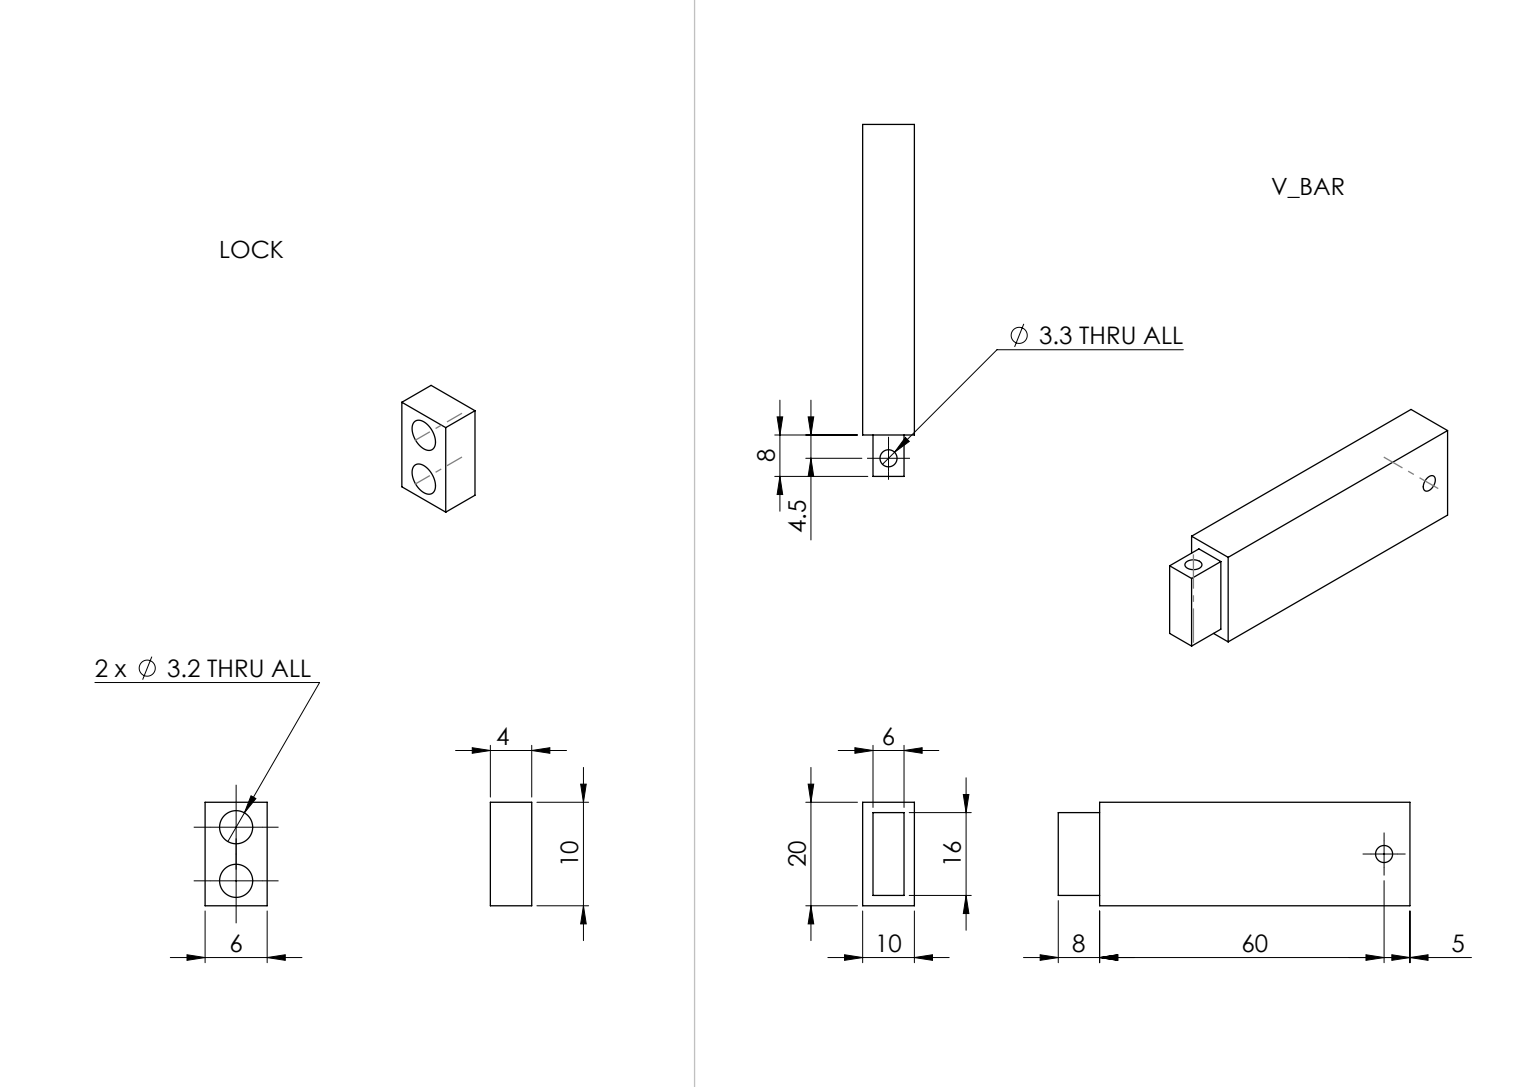
ISO-10303-21;
HEADER;
FILE_DESCRIPTION (('STEP AP214'),
    '1' );
FILE_NAME ('V_bar.step',
    '2026-10-08T12:12:07',
    ( '' ),
    ( '' ),
    'SwSTEP 2.0',
    'SolidWorks 2026',
    '' );
FILE_SCHEMA (( 'AUTOMOTIVE_DESIGN' ));
ENDSEC;

DATA;
#54=CARTESIAN_POINT ( 'NONE',  ( 55.00000000000000000, -8.000000000000001776, -4.499999999999986677 ) ) ;
#92=( NAMED_UNIT ( * ) PLANE_ANGLE_UNIT ( ) SI_UNIT ( $, .RADIAN. ) );
#93=AXIS2_PLACEMENT_3D ( 'NONE', #1716, #4922, #1673 ) ;
#102=VECTOR ( 'NONE', #7211, 1000.000000000000000 ) ;
#104=VECTOR ( 'NONE', #3751, 1000.000000000000000 ) ;
#145=LINE ( 'NONE', #2653, #909 ) ;
#163=DIRECTION ( 'NONE',  ( 0.000000000000000000, 1.000000000000000000, -0.000000000000000000 ) ) ;
#215=DIRECTION ( 'NONE',  ( 0.000000000000000000, 0.000000000000000000, 1.000000000000000000 ) ) ;
#229=ORIENTED_EDGE ( 'NONE', *, *, #6061, .F. ) ;
#234=LINE ( 'NONE', #6015, #2684 ) ;
#235=PLANE ( 'NONE',  #5820 ) ;
#258=DIRECTION ( 'NONE',  ( -0.000000000000000000, -1.000000000000000000, -0.000000000000000000 ) ) ;
#265=CARTESIAN_POINT ( 'NONE',  ( 60.00000000000000711, 9.332579536216795825E-15, 53.34999999999999432 ) ) ;
#266=CARTESIAN_POINT ( 'NONE',  ( 55.00000000000000000, 8.000000000000000000, -4.499999999999986677 ) ) ;
#270=CARTESIAN_POINT ( 'NONE',  ( 0.000000000000000000, 0.000000000000000000, 60.00000000000000000 ) ) ;
#293=ADVANCED_BREP_SHAPE_REPRESENTATION ( '', ( #1362, #1587 ), #1923 ) ;
#299=DIRECTION ( 'NONE',  ( 0.000000000000000000, 0.000000000000000000, -1.000000000000000000 ) ) ;
#302=FACE_BOUND ( 'NONE', #1666, .T. ) ;
#303=EDGE_CURVE ( 'NONE', #972, #4432, #3116, .T. ) ;
#319=LINE ( 'NONE', #2908, #3181 ) ;
#354=EDGE_CURVE ( 'NONE', #3615, #8148, #1959, .T. ) ;
#394=DIRECTION ( 'NONE',  ( 0.000000000000000000, 0.000000000000000000, 1.000000000000000000 ) ) ;
#407=DIRECTION ( 'NONE',  ( -0.000000000000000000, 1.000000000000000000, -0.000000000000000000 ) ) ;
#421=ORIENTED_EDGE ( 'NONE', *, *, #7234, .F. ) ;
#445=ADVANCED_FACE ( 'NONE', ( #302, #3325 ), #3433, .F. ) ;
#483=CARTESIAN_POINT ( 'NONE',  ( 50.00000000000000000, 9.332579536216795825E-15, 53.34999999999998010 ) ) ;
#539=CARTESIAN_POINT ( 'NONE',  ( 52.00000000000000711, -8.000000000000000000, -8.000000000000000000 ) ) ;
#555=CARTESIAN_POINT ( 'NONE',  ( 60.00000000000000711, 9.332579536216795825E-15, 54.99999999999997868 ) ) ;
#556=EDGE_CURVE ( 'NONE', #3047, #4432, #4306, .T. ) ;
#577=FACE_OUTER_BOUND ( 'NONE', #3634, .T. ) ;
#584=ORIENTED_EDGE ( 'NONE', *, *, #7801, .T. ) ;
#599=( LENGTH_UNIT ( ) NAMED_UNIT ( * ) SI_UNIT ( .MILLI., .METRE. ) );
#603=EDGE_LOOP ( 'NONE', ( #3185, #4958, #6458, #2037 ) ) ;
#684=DIRECTION ( 'NONE',  ( 0.000000000000000000, -1.000000000000000000, 0.000000000000000000 ) ) ;
#712=DIRECTION ( 'NONE',  ( 1.000000000000000000, -0.000000000000000000, -0.000000000000000000 ) ) ;
#717=ORIENTED_EDGE ( 'NONE', *, *, #2095, .F. ) ;
#723=SURFACE_STYLE_USAGE ( .BOTH. , #1946 ) ;
#724=AXIS2_PLACEMENT_3D ( 'NONE', #6540, #847, #215 ) ;
#726=FACE_OUTER_BOUND ( 'NONE', #4926, .T. ) ;
#743=DIRECTION ( 'NONE',  ( 0.000000000000000000, 0.000000000000000000, 1.000000000000000000 ) ) ;
#748=ORIENTED_EDGE ( 'NONE', *, *, #354, .T. ) ;
#760=AXIS2_PLACEMENT_3D ( 'NONE', #3959, #712, #2125 ) ;
#787=CARTESIAN_POINT ( 'NONE',  ( 60.00000000000000711, -10.00000000000000000, 60.00000000000000000 ) ) ;
#817=ORIENTED_EDGE ( 'NONE', *, *, #1983, .F. ) ;
#847=DIRECTION ( 'NONE',  ( 0.000000000000000000, 1.000000000000000000, -0.000000000000000000 ) ) ;
#879=CARTESIAN_POINT ( 'NONE',  ( 50.00000000000000000, -10.00000000000000000, 60.00000000000000000 ) ) ;
#897=EDGE_LOOP ( 'NONE', ( #2622, #3835 ) ) ;
#909=VECTOR ( 'NONE', #6307, 1000.000000000000000 ) ;
#916=VECTOR ( 'NONE', #3282, 1000.000000000000000 ) ;
#925=AXIS2_PLACEMENT_3D ( 'NONE', #4433, #1231, #6296 ) ;
#931=VERTEX_POINT ( 'NONE', #6838 ) ;
#942=EDGE_CURVE ( 'NONE', #8148, #2793, #145, .T. ) ;
#962=LINE ( 'NONE', #4254, #7895 ) ;
#972=VERTEX_POINT ( 'NONE', #2032 ) ;
#981=ORIENTED_EDGE ( 'NONE', *, *, #3877, .F. ) ;
#990=CARTESIAN_POINT ( 'NONE',  ( 50.00000000000000000, 10.00000000000000000, 60.00000000000000000 ) ) ;
#996=DIRECTION ( 'NONE',  ( 0.000000000000000000, 0.000000000000000000, -1.000000000000000000 ) ) ;
#1018=LINE ( 'NONE', #5356, #7945 ) ;
#1027=DIRECTION ( 'NONE',  ( 1.000000000000000000, 0.000000000000000000, 0.000000000000000000 ) ) ;
#1030=LINE ( 'NONE', #990, #5691 ) ;
#1046=ORIENTED_EDGE ( 'NONE', *, *, #7455, .T. ) ;
#1064=DIRECTION ( 'NONE',  ( 1.000000000000000000, 0.000000000000000000, 0.000000000000000000 ) ) ;
#1092=DIRECTION ( 'NONE',  ( 1.000000000000000000, -0.000000000000000000, -0.000000000000000000 ) ) ;
#1093=FILL_AREA_STYLE_COLOUR ( '', #7081 ) ;
#1106=STYLED_ITEM ( 'NONE', ( #5550 ), #293 ) ;
#1118=LINE ( 'NONE', #539, #4085 ) ;
#1136=( NAMED_UNIT ( * ) SI_UNIT ( $, .STERADIAN. ) SOLID_ANGLE_UNIT ( ) );
#1147=ORIENTED_EDGE ( 'NONE', *, *, #5934, .F. ) ;
#1162=ORIENTED_EDGE ( 'NONE', *, *, #6234, .T. ) ;
#1174=ORIENTED_EDGE ( 'NONE', *, *, #1998, .F. ) ;
#1193=AXIS2_PLACEMENT_3D ( 'NONE', #1933, #5753, #5667 ) ;
#1200=LINE ( 'NONE', #6929, #6572 ) ;
#1229=FILL_AREA_STYLE ('',( #1093 ) ) ;
#1231=DIRECTION ( 'NONE',  ( 1.000000000000000000, -0.000000000000000000, -0.000000000000000000 ) ) ;
#1248=DIRECTION ( 'NONE',  ( 0.000000000000000000, 1.000000000000000000, -0.000000000000000000 ) ) ;
#1277=EDGE_CURVE ( 'NONE', #5489, #8148, #8025, .T. ) ;
#1362=MANIFOLD_SOLID_BREP ( 'Tap Drill for M4 Tap2', #4092 ) ;
#1364=DIRECTION ( 'NONE',  ( 0.000000000000000000, -0.000000000000000000, 1.000000000000000000 ) ) ;
#1365=DIRECTION ( 'NONE',  ( 0.000000000000000000, 0.000000000000000000, 1.000000000000000000 ) ) ;
#1369=EDGE_CURVE ( 'NONE', #6012, #4327, #5321, .T. ) ;
#1390=FACE_BOUND ( 'NONE', #897, .T. ) ;
#1407=ORIENTED_EDGE ( 'NONE', *, *, #303, .F. ) ;
#1469=EDGE_CURVE ( 'NONE', #3630, #3047, #962, .T. ) ;
#1475=FACE_OUTER_BOUND ( 'NONE', #3870, .T. ) ;
#1486=DIRECTION ( 'NONE',  ( -1.000000000000000000, 0.000000000000000000, 0.000000000000000000 ) ) ;
#1507=CARTESIAN_POINT ( 'NONE',  ( 58.00000000000000000, -8.000000000000000000, 0.000000000000000000 ) ) ;
#1530=EDGE_LOOP ( 'NONE', ( #6903, #2912, #2180, #3251 ) ) ;
#1560=DIRECTION ( 'NONE',  ( 0.000000000000000000, 0.000000000000000000, 1.000000000000000000 ) ) ;
#1567=FACE_OUTER_BOUND ( 'NONE', #6558, .T. ) ;
#1587=AXIS2_PLACEMENT_3D ( 'NONE', #3942, #5152, #6454 ) ;
#1607=LINE ( 'NONE', #7781, #1909 ) ;
#1626=DIRECTION ( 'NONE',  ( -0.000000000000000000, -0.000000000000000000, -1.000000000000000000 ) ) ;
#1631=EDGE_CURVE ( 'NONE', #3615, #6597, #2117, .T. ) ;
#1658=CYLINDRICAL_SURFACE ( 'NONE', #5801, 1.649999999999995248 ) ;
#1663=CARTESIAN_POINT ( 'NONE',  ( 55.00000000000000000, 10.00000000000000000, -4.499999999999986677 ) ) ;
#1666=EDGE_LOOP ( 'NONE', ( #5675, #5495 ) ) ;
#1673=DIRECTION ( 'NONE',  ( 1.000000000000000000, 0.000000000000000000, -0.000000000000000000 ) ) ;
#1676=ORIENTED_EDGE ( 'NONE', *, *, #1631, .F. ) ;
#1704=VECTOR ( 'NONE', #6343, 1000.000000000000000 ) ;
#1709=VECTOR ( 'NONE', #7695, 1000.000000000000000 ) ;
#1714=ADVANCED_FACE ( 'NONE', ( #7304 ), #5443, .T. ) ;
#1716=CARTESIAN_POINT ( 'NONE',  ( 0.000000000000000000, 0.000000000000000000, -8.000000000000000000 ) ) ;
#1750=EDGE_CURVE ( 'NONE', #3287, #2510, #6633, .T. ) ;
#1753=CARTESIAN_POINT ( 'NONE',  ( 52.00000000000000711, -8.000000000000000000, -8.000000000000000000 ) ) ;
#1770=EDGE_CURVE ( 'NONE', #3287, #5411, #4813, .T. ) ;
#1785=ADVANCED_FACE ( 'NONE', ( #7339 ), #1658, .F. ) ;
#1828=EDGE_LOOP ( 'NONE', ( #2953, #1676, #6166, #1174 ) ) ;
#1840=ORIENTED_EDGE ( 'NONE', *, *, #1277, .F. ) ;
#1843=CARTESIAN_POINT ( 'NONE',  ( 58.00000000000000000, -8.000000000000000000, 0.000000000000000000 ) ) ;
#1876=PRODUCT ( 'V_bar', 'V_bar', '', ( #2708 ) ) ;
#1903=DIRECTION ( 'NONE',  ( 0.000000000000000000, 0.000000000000000000, -1.000000000000000000 ) ) ;
#1907=PRESENTATION_STYLE_ASSIGNMENT (( #723 ) ) ;
#1909=VECTOR ( 'NONE', #6570, 1000.000000000000000 ) ;
#1923=( GEOMETRIC_REPRESENTATION_CONTEXT ( 3 ) GLOBAL_UNCERTAINTY_ASSIGNED_CONTEXT ( ( #7447 ) ) GLOBAL_UNIT_ASSIGNED_CONTEXT ( ( #6567, #2842, #3508 ) ) REPRESENTATION_CONTEXT ( 'NONE', 'WORKASPACE' ) );
#1931=EDGE_LOOP ( 'NONE', ( #7376, #6911 ) ) ;
#1933=CARTESIAN_POINT ( 'NONE',  ( 60.00000000000000711, 10.00000000000000000, 60.00000000000000000 ) ) ;
#1946=SURFACE_SIDE_STYLE ('',( #6452 ) ) ;
#1956=VECTOR ( 'NONE', #6675, 1000.000000000000000 ) ;
#1959=LINE ( 'NONE', #2038, #2174 ) ;
#1983=EDGE_CURVE ( 'NONE', #4068, #4327, #1200, .T. ) ;
#1994=AXIS2_PLACEMENT_3D ( 'NONE', #7084, #1364, #5033 ) ;
#1998=EDGE_CURVE ( 'NONE', #7134, #931, #5155, .T. ) ;
#2032=CARTESIAN_POINT ( 'NONE',  ( 55.00000000000000000, -8.000000000000001776, -6.149999999999981704 ) ) ;
#2037=ORIENTED_EDGE ( 'NONE', *, *, #6966, .T. ) ;
#2038=CARTESIAN_POINT ( 'NONE',  ( 52.00000000000000711, 8.000000000000000000, -8.000000000000000000 ) ) ;
#2086=CARTESIAN_POINT ( 'NONE',  ( 50.00000000000000000, -10.00000000000000000, 60.00000000000000000 ) ) ;
#2090=ORIENTED_EDGE ( 'NONE', *, *, #1631, .T. ) ;
#2095=EDGE_CURVE ( 'NONE', #2510, #6841, #4753, .T. ) ;
#2111=AXIS2_PLACEMENT_3D ( 'NONE', #555, #3635, #6698 ) ;
#2117=LINE ( 'NONE', #5245, #3398 ) ;
#2121=CIRCLE ( 'NONE', #3049, 1.649999999999998579 ) ;
#2125=DIRECTION ( 'NONE',  ( 0.000000000000000000, 0.000000000000000000, -1.000000000000000000 ) ) ;
#2137=EDGE_CURVE ( 'NONE', #6584, #6037, #1607, .T. ) ;
#2174=VECTOR ( 'NONE', #5693, 1000.000000000000000 ) ;
#2180=ORIENTED_EDGE ( 'NONE', *, *, #5385, .T. ) ;
#2191=CARTESIAN_POINT ( 'NONE',  ( 55.00000000000000000, 10.00000000000000000, -4.499999999999986677 ) ) ;
#2192=EDGE_CURVE ( 'NONE', #4327, #6012, #4142, .T. ) ;
#2197=CARTESIAN_POINT ( 'NONE',  ( 50.00000000000000000, 10.00000000000000000, 60.00000000000000000 ) ) ;
#2281=ORIENTED_EDGE ( 'NONE', *, *, #4024, .T. ) ;
#2327=ORIENTED_EDGE ( 'NONE', *, *, #6061, .T. ) ;
#2335=AXIS2_PLACEMENT_3D ( 'NONE', #270, #7961, #4065 ) ;
#2360=PLANE ( 'NONE',  #6129 ) ;
#2361=VECTOR ( 'NONE', #7420, 1000.000000000000000 ) ;
#2362=LINE ( 'NONE', #3529, #7673 ) ;
#2376=PLANE ( 'NONE',  #93 ) ;
#2380=VECTOR ( 'NONE', #2938, 1000.000000000000000 ) ;
#2390=CARTESIAN_POINT ( 'NONE',  ( 58.00000000000000000, -8.000000000000000000, -8.000000000000000000 ) ) ;
#2423=CARTESIAN_POINT ( 'NONE',  ( 52.00000000000000711, 8.000000000000000000, -8.000000000000000000 ) ) ;
#2453=CARTESIAN_POINT ( 'NONE',  ( 60.00000000000000711, -10.00000000000000000, 0.000000000000000000 ) ) ;
#2466=ORIENTED_EDGE ( 'NONE', *, *, #3877, .T. ) ;
#2502=ORIENTED_EDGE ( 'NONE', *, *, #942, .F. ) ;
#2510=VERTEX_POINT ( 'NONE', #2197 ) ;
#2520=EDGE_CURVE ( 'NONE', #2793, #5096, #234, .T. ) ;
#2537=COLOUR_RGB ( '', 0.66274510, 0.83137255, 0.94901961) ;
#2592=ADVANCED_FACE ( 'NONE', ( #7222 ), #5451, .F. ) ;
#2596=AXIS2_PLACEMENT_3D ( 'NONE', #3358, #1486, #1560 ) ;
#2601=ORIENTED_EDGE ( 'NONE', *, *, #303, .T. ) ;
#2622=ORIENTED_EDGE ( 'NONE', *, *, #7234, .T. ) ;
#2653=CARTESIAN_POINT ( 'NONE',  ( 52.00000000000000711, 8.000000000000000000, 0.000000000000000000 ) ) ;
#2657=CARTESIAN_POINT ( 'NONE',  ( 55.00000000000000000, 10.00000000000000000, -6.149999999999981704 ) ) ;
#2662=LINE ( 'NONE', #2696, #916 ) ;
#2681=ADVANCED_FACE ( 'NONE', ( #6935, #577 ), #2360, .T. ) ;
#2684=VECTOR ( 'NONE', #1027, 1000.000000000000000 ) ;
#2696=CARTESIAN_POINT ( 'NONE',  ( 60.00000000000000711, -10.00000000000000000, 0.000000000000000000 ) ) ;
#2708=PRODUCT_CONTEXT ( 'NONE', #3818, 'mechanical' ) ;
#2721=ORIENTED_EDGE ( 'NONE', *, *, #4889, .F. ) ;
#2750=CARTESIAN_POINT ( 'NONE',  ( 60.00000000000000711, 10.00000000000000000, 60.00000000000000000 ) ) ;
#2782=EDGE_LOOP ( 'NONE', ( #7659, #7484, #6677, #6945 ) ) ;
#2793=VERTEX_POINT ( 'NONE', #4566 ) ;
#2814=DIRECTION ( 'NONE',  ( 0.000000000000000000, 1.000000000000000000, -0.000000000000000000 ) ) ;
#2819=DIRECTION ( 'NONE',  ( -0.000000000000000000, -0.000000000000000000, -1.000000000000000000 ) ) ;
#2842=( NAMED_UNIT ( * ) PLANE_ANGLE_UNIT ( ) SI_UNIT ( $, .RADIAN. ) );
#2862=EDGE_CURVE ( 'NONE', #3630, #972, #6048, .T. ) ;
#2908=CARTESIAN_POINT ( 'NONE',  ( 60.00000000000000711, -10.00000000000000000, 60.00000000000000000 ) ) ;
#2912=ORIENTED_EDGE ( 'NONE', *, *, #2520, .T. ) ;
#2938=DIRECTION ( 'NONE',  ( 0.000000000000000000, 0.000000000000000000, 1.000000000000000000 ) ) ;
#2947=DIRECTION ( 'NONE',  ( 0.000000000000000000, 0.000000000000000000, 1.000000000000000000 ) ) ;
#2953=ORIENTED_EDGE ( 'NONE', *, *, #7801, .F. ) ;
#2963=ORIENTED_EDGE ( 'NONE', *, *, #5726, .T. ) ;
#2995=ORIENTED_EDGE ( 'NONE', *, *, #1770, .T. ) ;
#2997=VECTOR ( 'NONE', #2819, 1000.000000000000000 ) ;
#3037=EDGE_LOOP ( 'NONE', ( #7751, #2601, #7521, #5999 ) ) ;
#3047=VERTEX_POINT ( 'NONE', #4762 ) ;
#3049=AXIS2_PLACEMENT_3D ( 'NONE', #5012, #1092, #6744 ) ;
#3056=VECTOR ( 'NONE', #7356, 1000.000000000000000 ) ;
#3061=STYLED_ITEM ( 'NONE', ( #1907 ), #1362 ) ;
#3064=CARTESIAN_POINT ( 'NONE',  ( 50.00000000000000000, -10.00000000000000000, 60.00000000000000000 ) ) ;
#3116=LINE ( 'NONE', #2657, #7090 ) ;
#3142=SURFACE_SIDE_STYLE ('',( #4340 ) ) ;
#3181=VECTOR ( 'NONE', #8044, 1000.000000000000000 ) ;
#3185=ORIENTED_EDGE ( 'NONE', *, *, #5385, .F. ) ;
#3228=ORIENTED_EDGE ( 'NONE', *, *, #1770, .F. ) ;
#3251=ORIENTED_EDGE ( 'NONE', *, *, #1277, .T. ) ;
#3258=PLANE ( 'NONE',  #3975 ) ;
#3282=DIRECTION ( 'NONE',  ( 1.000000000000000000, -0.000000000000000000, -0.000000000000000000 ) ) ;
#3287=VERTEX_POINT ( 'NONE', #2750 ) ;
#3325=FACE_OUTER_BOUND ( 'NONE', #4284, .T. ) ;
#3352=CARTESIAN_POINT ( 'NONE',  ( 58.00000000000000000, -8.000000000000000000, -8.000000000000000000 ) ) ;
#3358=CARTESIAN_POINT ( 'NONE',  ( 60.00000000000000711, -10.00000000000000000, 60.00000000000000000 ) ) ;
#3370=FACE_OUTER_BOUND ( 'NONE', #6792, .T. ) ;
#3385=ADVANCED_FACE ( 'NONE', ( #3627 ), #2376, .F. ) ;
#3398=VECTOR ( 'NONE', #6247, 1000.000000000000000 ) ;
#3403=AXIS2_PLACEMENT_3D ( 'NONE', #6507, #4486, #7720 ) ;
#3423=CYLINDRICAL_SURFACE ( 'NONE', #2111, 1.649999999999991696 ) ;
#3433=PLANE ( 'NONE',  #2596 ) ;
#3440=AXIS2_PLACEMENT_3D ( 'NONE', #266, #2814, #7869 ) ;
#3449=ORIENTED_EDGE ( 'NONE', *, *, #1469, .T. ) ;
#3485=CARTESIAN_POINT ( 'NONE',  ( 60.00000000000000711, 10.00000000000000000, 60.00000000000000000 ) ) ;
#3508=( NAMED_UNIT ( * ) SI_UNIT ( $, .STERADIAN. ) SOLID_ANGLE_UNIT ( ) );
#3529=CARTESIAN_POINT ( 'NONE',  ( 60.00000000000000711, 10.00000000000000000, 0.000000000000000000 ) ) ;
#3537=FACE_OUTER_BOUND ( 'NONE', #7838, .T. ) ;
#3560=DIRECTION ( 'NONE',  ( -0.000000000000000000, -0.000000000000000000, -1.000000000000000000 ) ) ;
#3568=ORIENTED_EDGE ( 'NONE', *, *, #4117, .F. ) ;
#3581=ORIENTED_EDGE ( 'NONE', *, *, #5633, .F. ) ;
#3615=VERTEX_POINT ( 'NONE', #2423 ) ;
#3627=FACE_OUTER_BOUND ( 'NONE', #1828, .T. ) ;
#3630=VERTEX_POINT ( 'NONE', #7580 ) ;
#3634=EDGE_LOOP ( 'NONE', ( #1840, #6249, #1046, #748 ) ) ;
#3635=DIRECTION ( 'NONE',  ( 1.000000000000000000, -0.000000000000000000, -0.000000000000000000 ) ) ;
#3719=ADVANCED_FACE ( 'NONE', ( #1390, #3370 ), #3258, .F. ) ;
#3736=VERTEX_POINT ( 'NONE', #5866 ) ;
#3751=DIRECTION ( 'NONE',  ( 0.000000000000000000, 1.000000000000000000, 0.000000000000000000 ) ) ;
#3794=ORIENTED_EDGE ( 'NONE', *, *, #5726, .F. ) ;
#3806=ORIENTED_EDGE ( 'NONE', *, *, #1369, .T. ) ;
#3808=EDGE_CURVE ( 'NONE', #4068, #4539, #6593, .T. ) ;
#3818=APPLICATION_CONTEXT ( 'automotive_design' ) ;
#3833=LINE ( 'NONE', #2453, #104 ) ;
#3835=ORIENTED_EDGE ( 'NONE', *, *, #3808, .T. ) ;
#3870=EDGE_LOOP ( 'NONE', ( #7901, #5941, #584, #5279 ) ) ;
#3877=EDGE_CURVE ( 'NONE', #2510, #6584, #1030, .T. ) ;
#3936=FILL_AREA_STYLE ('',( #7628 ) ) ;
#3942=CARTESIAN_POINT ( 'NONE',  ( 0.000000000000000000, 0.000000000000000000, 0.000000000000000000 ) ) ;
#3959=CARTESIAN_POINT ( 'NONE',  ( 50.00000000000000000, 9.332579536216795825E-15, 54.99999999999997868 ) ) ;
#3975=AXIS2_PLACEMENT_3D ( 'NONE', #2086, #7144, #6554 ) ;
#3989=AXIS2_PLACEMENT_3D ( 'NONE', #4014, #5907, #996 ) ;
#4011=ORIENTED_EDGE ( 'NONE', *, *, #2095, .T. ) ;
#4014=CARTESIAN_POINT ( 'NONE',  ( 60.00000000000000711, 9.332579536216795825E-15, 54.99999999999997868 ) ) ;
#4024=EDGE_CURVE ( 'NONE', #6597, #2793, #1118, .T. ) ;
#4033=DIRECTION ( 'NONE',  ( -0.000000000000000000, 1.000000000000000000, -0.000000000000000000 ) ) ;
#4052=CARTESIAN_POINT ( 'NONE',  ( 58.00000000000000000, -8.000000000000000000, -8.000000000000000000 ) ) ;
#4065=DIRECTION ( 'NONE',  ( 1.000000000000000000, 0.000000000000000000, -0.000000000000000000 ) ) ;
#4067=ORIENTED_EDGE ( 'NONE', *, *, #5635, .T. ) ;
#4068=VERTEX_POINT ( 'NONE', #6510 ) ;
#4085=VECTOR ( 'NONE', #6181, 1000.000000000000000 ) ;
#4092=CLOSED_SHELL ( 'NONE', ( #7407, #2592, #445, #5310, #3719, #5469, #1714, #4442, #7344, #4209, #2681, #7194, #3385, #1785, #4715 ) ) ;
#4104=DIRECTION ( 'NONE',  ( -1.000000000000000000, 0.000000000000000000, 0.000000000000000000 ) ) ;
#4117=EDGE_CURVE ( 'NONE', #6037, #5610, #2662, .T. ) ;
#4125=FACE_OUTER_BOUND ( 'NONE', #2782, .T. ) ;
#4142=CIRCLE ( 'NONE', #7324, 1.649999999999984812 ) ;
#4154=DIRECTION ( 'NONE',  ( -0.000000000000000000, 1.000000000000000000, -0.000000000000000000 ) ) ;
#4199=EDGE_LOOP ( 'NONE', ( #6739, #2721 ) ) ;
#4204=EDGE_CURVE ( 'NONE', #6841, #6037, #1018, .T. ) ;
#4209=ADVANCED_FACE ( 'NONE', ( #1567 ), #4766, .T. ) ;
#4221=CARTESIAN_POINT ( 'NONE',  ( 50.00000000000000000, -10.00000000000000000, 0.000000000000000000 ) ) ;
#4254=CARTESIAN_POINT ( 'NONE',  ( 55.00000000000000000, 10.00000000000000000, -2.849999999999991651 ) ) ;
#4257=EDGE_LOOP ( 'NONE', ( #1407, #7999, #3449, #8061 ) ) ;
#4284=EDGE_LOOP ( 'NONE', ( #2963, #3228, #229, #6053 ) ) ;
#4306=CIRCLE ( 'NONE', #724, 1.649999999999995248 ) ;
#4313=PRODUCT_DEFINITION_SHAPE ( 'NONE', 'NONE',  #6186 ) ;
#4327=VERTEX_POINT ( 'NONE', #7857 ) ;
#4340=SURFACE_STYLE_FILL_AREA ( #1229 ) ;
#4342=CARTESIAN_POINT ( 'NONE',  ( 58.00000000000000000, 8.000000000000000000, 0.000000000000000000 ) ) ;
#4380=AXIS2_PLACEMENT_3D ( 'NONE', #2390, #7456, #4838 ) ;
#4391=SURFACE_STYLE_USAGE ( .BOTH. , #3142 ) ;
#4400=LINE ( 'NONE', #7548, #1704 ) ;
#4417=PRODUCT_DEFINITION_CONTEXT ( 'detailed design', #4503, 'design' ) ;
#4432=VERTEX_POINT ( 'NONE', #6391 ) ;
#4433=CARTESIAN_POINT ( 'NONE',  ( 60.00000000000000711, 9.332579536216795825E-15, 54.99999999999997868 ) ) ;
#4442=ADVANCED_FACE ( 'NONE', ( #5572, #726 ), #6270, .F. ) ;
#4449=DIRECTION ( 'NONE',  ( 0.000000000000000000, 0.000000000000000000, 1.000000000000000000 ) ) ;
#4477=CARTESIAN_POINT ( 'NONE',  ( 58.00000000000000000, 8.000000000000000000, -8.000000000000000000 ) ) ;
#4486=DIRECTION ( 'NONE',  ( 0.000000000000000000, -1.000000000000000000, 0.000000000000000000 ) ) ;
#4503=APPLICATION_CONTEXT ( 'automotive_design' ) ;
#4539=VERTEX_POINT ( 'NONE', #483 ) ;
#4542=ORIENTED_EDGE ( 'NONE', *, *, #1750, .F. ) ;
#4566=CARTESIAN_POINT ( 'NONE',  ( 52.00000000000000711, -8.000000000000000000, 0.000000000000000000 ) ) ;
#4632=CIRCLE ( 'NONE', #3440, 1.649999999999995248 ) ;
#4686=PRODUCT_DEFINITION_FORMATION_WITH_SPECIFIED_SOURCE ( 'ANY', '', #1876, .NOT_KNOWN. ) ;
#4690=EDGE_LOOP ( 'NONE', ( #2327, #7439, #4011, #4736 ) ) ;
#4715=ADVANCED_FACE ( 'NONE', ( #6564 ), #3423, .F. ) ;
#4720=LINE ( 'NONE', #4848, #2380 ) ;
#4724=DIRECTION ( 'NONE',  ( 0.000000000000000000, 0.000000000000000000, 1.000000000000000000 ) ) ;
#4736=ORIENTED_EDGE ( 'NONE', *, *, #5934, .T. ) ;
#4738=DIRECTION ( 'NONE',  ( 0.000000000000000000, -0.000000000000000000, -1.000000000000000000 ) ) ;
#4753=LINE ( 'NONE', #879, #5483 ) ;
#4762=CARTESIAN_POINT ( 'NONE',  ( 55.00000000000000000, 8.000000000000000000, -2.849999999999991651 ) ) ;
#4765=CARTESIAN_POINT ( 'NONE',  ( 52.00000000000000711, -8.000000000000000000, -8.000000000000000000 ) ) ;
#4766=PLANE ( 'NONE',  #6496 ) ;
#4779=DIRECTION ( 'NONE',  ( -1.000000000000000000, 0.000000000000000000, 0.000000000000000000 ) ) ;
#4813=LINE ( 'NONE', #3485, #2997 ) ;
#4823=MECHANICAL_DESIGN_GEOMETRIC_PRESENTATION_REPRESENTATION('',(#1106),#6284);
#4831=CARTESIAN_POINT ( 'NONE',  ( 58.00000000000000000, 8.000000000000000000, -8.000000000000000000 ) ) ;
#4838=DIRECTION ( 'NONE',  ( 0.000000000000000000, 0.000000000000000000, -1.000000000000000000 ) ) ;
#4848=CARTESIAN_POINT ( 'NONE',  ( 58.00000000000000000, -8.000000000000000000, -8.000000000000000000 ) ) ;
#4880=PLANE ( 'NONE',  #4380 ) ;
#4889=EDGE_CURVE ( 'NONE', #972, #3630, #6089, .T. ) ;
#4908=CARTESIAN_POINT ( 'NONE',  ( 60.00000000000000711, -10.00000000000000000, 0.000000000000000000 ) ) ;
#4922=DIRECTION ( 'NONE',  ( 0.000000000000000000, 0.000000000000000000, 1.000000000000000000 ) ) ;
#4926=EDGE_LOOP ( 'NONE', ( #3794, #3568, #5584, #6751 ) ) ;
#4958=ORIENTED_EDGE ( 'NONE', *, *, #7859, .F. ) ;
#4974=( NAMED_UNIT ( * ) PLANE_ANGLE_UNIT ( ) SI_UNIT ( $, .RADIAN. ) );
#5012=CARTESIAN_POINT ( 'NONE',  ( 50.00000000000000000, 9.332579536216795825E-15, 54.99999999999997868 ) ) ;
#5017=ORIENTED_EDGE ( 'NONE', *, *, #354, .F. ) ;
#5033=DIRECTION ( 'NONE',  ( 1.000000000000000000, 0.000000000000000000, -0.000000000000000000 ) ) ;
#5065=FACE_BOUND ( 'NONE', #4199, .T. ) ;
#5096=VERTEX_POINT ( 'NONE', #1507 ) ;
#5152=DIRECTION ( 'NONE',  ( 0.000000000000000000, 0.000000000000000000, 1.000000000000000000 ) ) ;
#5155=LINE ( 'NONE', #3352, #5673 ) ;
#5199=DIRECTION ( 'NONE',  ( 1.000000000000000000, -0.000000000000000000, -0.000000000000000000 ) ) ;
#5245=CARTESIAN_POINT ( 'NONE',  ( 52.00000000000000711, 8.000000000000000000, -8.000000000000000000 ) ) ;
#5279=ORIENTED_EDGE ( 'NONE', *, *, #7859, .T. ) ;
#5309=CARTESIAN_POINT ( 'NONE',  ( 60.00000000000000711, 9.332579536216795825E-15, 54.99999999999997868 ) ) ;
#5310=ADVANCED_FACE ( 'NONE', ( #3537 ), #5710, .F. ) ;
#5321=CIRCLE ( 'NONE', #925, 1.649999999999984812 ) ;
#5356=CARTESIAN_POINT ( 'NONE',  ( 50.00000000000000000, -10.00000000000000000, 60.00000000000000000 ) ) ;
#5385=EDGE_CURVE ( 'NONE', #5096, #5489, #7577, .T. ) ;
#5411=VERTEX_POINT ( 'NONE', #6242 ) ;
#5413=DIRECTION ( 'NONE',  ( 0.000000000000000000, -1.000000000000000000, 0.000000000000000000 ) ) ;
#5443=PLANE ( 'NONE',  #2335 ) ;
#5451=CYLINDRICAL_SURFACE ( 'NONE', #7603, 1.649999999999995248 ) ;
#5454=( GEOMETRIC_REPRESENTATION_CONTEXT ( 3 ) GLOBAL_UNCERTAINTY_ASSIGNED_CONTEXT ( ( #7942 ) ) GLOBAL_UNIT_ASSIGNED_CONTEXT ( ( #5802, #92, #5765 ) ) REPRESENTATION_CONTEXT ( 'NONE', 'WORKASPACE' ) );
#5469=ADVANCED_FACE ( 'NONE', ( #5865 ), #235, .F. ) ;
#5483=VECTOR ( 'NONE', #258, 1000.000000000000000 ) ;
#5487=CARTESIAN_POINT ( 'NONE',  ( 60.00000000000000711, 10.00000000000000000, 60.00000000000000000 ) ) ;
#5489=VERTEX_POINT ( 'NONE', #7762 ) ;
#5495=ORIENTED_EDGE ( 'NONE', *, *, #2192, .F. ) ;
#5518=LINE ( 'NONE', #4765, #6908 ) ;
#5550=PRESENTATION_STYLE_ASSIGNMENT (( #4391 ) ) ;
#5572=FACE_BOUND ( 'NONE', #1530, .T. ) ;
#5584=ORIENTED_EDGE ( 'NONE', *, *, #2137, .F. ) ;
#5597=FACE_OUTER_BOUND ( 'NONE', #603, .T. ) ;
#5610=VERTEX_POINT ( 'NONE', #4908 ) ;
#5616=CARTESIAN_POINT ( 'NONE',  ( 58.00000000000000000, 8.000000000000000000, -8.000000000000000000 ) ) ;
#5633=EDGE_CURVE ( 'NONE', #3736, #5610, #319, .T. ) ;
#5635=EDGE_CURVE ( 'NONE', #5411, #6584, #2362, .T. ) ;
#5667=DIRECTION ( 'NONE',  ( 0.000000000000000000, -0.000000000000000000, -1.000000000000000000 ) ) ;
#5673=VECTOR ( 'NONE', #7007, 1000.000000000000000 ) ;
#5675=ORIENTED_EDGE ( 'NONE', *, *, #1369, .F. ) ;
#5691=VECTOR ( 'NONE', #1626, 1000.000000000000000 ) ;
#5693=DIRECTION ( 'NONE',  ( 0.000000000000000000, 0.000000000000000000, 1.000000000000000000 ) ) ;
#5710=PLANE ( 'NONE',  #1193 ) ;
#5726=EDGE_CURVE ( 'NONE', #5610, #5411, #3833, .T. ) ;
#5753=DIRECTION ( 'NONE',  ( 0.000000000000000000, -1.000000000000000000, 0.000000000000000000 ) ) ;
#5765=( NAMED_UNIT ( * ) SI_UNIT ( $, .STERADIAN. ) SOLID_ANGLE_UNIT ( ) );
#5801=AXIS2_PLACEMENT_3D ( 'NONE', #2191, #4033, #4724 ) ;
#5802=( LENGTH_UNIT ( ) NAMED_UNIT ( * ) SI_UNIT ( .MILLI., .METRE. ) );
#5820=AXIS2_PLACEMENT_3D ( 'NONE', #787, #163, #743 ) ;
#5843=VECTOR ( 'NONE', #1365, 1000.000000000000000 ) ;
#5865=FACE_OUTER_BOUND ( 'NONE', #6352, .T. ) ;
#5866=CARTESIAN_POINT ( 'NONE',  ( 60.00000000000000711, -10.00000000000000000, 60.00000000000000000 ) ) ;
#5872=LINE ( 'NONE', #4831, #3056 ) ;
#5907=DIRECTION ( 'NONE',  ( 1.000000000000000000, -0.000000000000000000, -0.000000000000000000 ) ) ;
#5915=CARTESIAN_POINT ( 'NONE',  ( 52.00000000000000711, 8.000000000000000000, 0.000000000000000000 ) ) ;
#5934=EDGE_CURVE ( 'NONE', #6841, #3736, #6578, .T. ) ;
#5941=ORIENTED_EDGE ( 'NONE', *, *, #4024, .F. ) ;
#5960=ORIENTED_EDGE ( 'NONE', *, *, #4204, .T. ) ;
#5999=ORIENTED_EDGE ( 'NONE', *, *, #1469, .F. ) ;
#6012=VERTEX_POINT ( 'NONE', #265 ) ;
#6015=CARTESIAN_POINT ( 'NONE',  ( 52.00000000000000711, -8.000000000000000000, 0.000000000000000000 ) ) ;
#6037=VERTEX_POINT ( 'NONE', #4221 ) ;
#6048=CIRCLE ( 'NONE', #3403, 1.649999999999995248 ) ;
#6053=ORIENTED_EDGE ( 'NONE', *, *, #5633, .T. ) ;
#6061=EDGE_CURVE ( 'NONE', #3736, #3287, #7868, .T. ) ;
#6089=CIRCLE ( 'NONE', #6233, 1.649999999999995248 ) ;
#6092=CARTESIAN_POINT ( 'NONE',  ( 52.00000000000000711, 8.000000000000000000, -8.000000000000000000 ) ) ;
#6129=AXIS2_PLACEMENT_3D ( 'NONE', #5616, #1248, #4449 ) ;
#6166=ORIENTED_EDGE ( 'NONE', *, *, #7455, .F. ) ;
#6181=DIRECTION ( 'NONE',  ( 0.000000000000000000, 0.000000000000000000, 1.000000000000000000 ) ) ;
#6186=PRODUCT_DEFINITION ( 'UNKNOWN', '', #4686, #4417 ) ;
#6233=AXIS2_PLACEMENT_3D ( 'NONE', #54, #684, #1903 ) ;
#6234=EDGE_CURVE ( 'NONE', #4539, #6012, #4400, .T. ) ;
#6235=AXIS2_PLACEMENT_3D ( 'NONE', #7193, #5413, #4738 ) ;
#6242=CARTESIAN_POINT ( 'NONE',  ( 60.00000000000000711, 10.00000000000000000, 0.000000000000000000 ) ) ;
#6247=DIRECTION ( 'NONE',  ( 0.000000000000000000, -1.000000000000000000, 0.000000000000000000 ) ) ;
#6249=ORIENTED_EDGE ( 'NONE', *, *, #6966, .F. ) ;
#6270=PLANE ( 'NONE',  #1994 ) ;
#6284=( GEOMETRIC_REPRESENTATION_CONTEXT ( 3 ) GLOBAL_UNCERTAINTY_ASSIGNED_CONTEXT ( ( #6779 ) ) GLOBAL_UNIT_ASSIGNED_CONTEXT ( ( #599, #4974, #1136 ) ) REPRESENTATION_CONTEXT ( 'NONE', 'WORKASPACE' ) );
#6296=DIRECTION ( 'NONE',  ( 0.000000000000000000, 0.000000000000000000, -1.000000000000000000 ) ) ;
#6307=DIRECTION ( 'NONE',  ( 0.000000000000000000, -1.000000000000000000, 0.000000000000000000 ) ) ;
#6343=DIRECTION ( 'NONE',  ( 1.000000000000000000, -0.000000000000000000, -0.000000000000000000 ) ) ;
#6352=EDGE_LOOP ( 'NONE', ( #7738, #3581, #1147, #5960 ) ) ;
#6391=CARTESIAN_POINT ( 'NONE',  ( 55.00000000000000000, 8.000000000000000000, -6.149999999999981704 ) ) ;
#6452=SURFACE_STYLE_FILL_AREA ( #3936 ) ;
#6454=DIRECTION ( 'NONE',  ( 1.000000000000000000, 0.000000000000000000, 0.000000000000000000 ) ) ;
#6458=ORIENTED_EDGE ( 'NONE', *, *, #1998, .T. ) ;
#6496=AXIS2_PLACEMENT_3D ( 'NONE', #6092, #4104, #394 ) ;
#6507=CARTESIAN_POINT ( 'NONE',  ( 55.00000000000000000, -8.000000000000001776, -4.499999999999986677 ) ) ;
#6510=CARTESIAN_POINT ( 'NONE',  ( 50.00000000000000000, 9.534646258076108189E-15, 56.64999999999997726 ) ) ;
#6540=CARTESIAN_POINT ( 'NONE',  ( 55.00000000000000000, 8.000000000000000000, -4.499999999999986677 ) ) ;
#6554=DIRECTION ( 'NONE',  ( 0.000000000000000000, 0.000000000000000000, -1.000000000000000000 ) ) ;
#6558=EDGE_LOOP ( 'NONE', ( #2502, #5017, #2090, #2281 ) ) ;
#6564=FACE_OUTER_BOUND ( 'NONE', #7204, .T. ) ;
#6567=( LENGTH_UNIT ( ) NAMED_UNIT ( * ) SI_UNIT ( .MILLI., .METRE. ) );
#6570=DIRECTION ( 'NONE',  ( -0.000000000000000000, -1.000000000000000000, -0.000000000000000000 ) ) ;
#6572=VECTOR ( 'NONE', #5199, 1000.000000000000000 ) ;
#6578=LINE ( 'NONE', #7057, #102 ) ;
#6584=VERTEX_POINT ( 'NONE', #6973 ) ;
#6593=CIRCLE ( 'NONE', #760, 1.649999999999998579 ) ;
#6597=VERTEX_POINT ( 'NONE', #1753 ) ;
#6603=CYLINDRICAL_SURFACE ( 'NONE', #3989, 1.649999999999991696 ) ;
#6633=LINE ( 'NONE', #5487, #1956 ) ;
#6675=DIRECTION ( 'NONE',  ( -1.000000000000000000, 0.000000000000000000, 0.000000000000000000 ) ) ;
#6677=ORIENTED_EDGE ( 'NONE', *, *, #2192, .T. ) ;
#6698=DIRECTION ( 'NONE',  ( 0.000000000000000000, 0.000000000000000000, -1.000000000000000000 ) ) ;
#6739=ORIENTED_EDGE ( 'NONE', *, *, #2862, .F. ) ;
#6744=DIRECTION ( 'NONE',  ( 0.000000000000000000, 0.000000000000000000, -1.000000000000000000 ) ) ;
#6751=ORIENTED_EDGE ( 'NONE', *, *, #5635, .F. ) ;
#6779=UNCERTAINTY_MEASURE_WITH_UNIT (LENGTH_MEASURE( 1.000000000000000082E-05 ), #599, 'distance_accuracy_value', 'NONE');
#6792=EDGE_LOOP ( 'NONE', ( #7595, #8038, #717, #2466 ) ) ;
#6838=CARTESIAN_POINT ( 'NONE',  ( 58.00000000000000000, 8.000000000000000000, -8.000000000000000000 ) ) ;
#6841=VERTEX_POINT ( 'NONE', #3064 ) ;
#6903=ORIENTED_EDGE ( 'NONE', *, *, #942, .T. ) ;
#6908=VECTOR ( 'NONE', #1064, 1000.000000000000000 ) ;
#6911=ORIENTED_EDGE ( 'NONE', *, *, #7847, .F. ) ;
#6929=CARTESIAN_POINT ( 'NONE',  ( 60.00000000000000711, 9.534646258076108189E-15, 56.64999999999997016 ) ) ;
#6935=FACE_BOUND ( 'NONE', #1931, .T. ) ;
#6945=ORIENTED_EDGE ( 'NONE', *, *, #6234, .F. ) ;
#6959=SHAPE_REPRESENTATION_RELATIONSHIP ( 'NONE' , 'NONE' ,  #6987, #293 ) ;
#6966=EDGE_CURVE ( 'NONE', #931, #5489, #7632, .T. ) ;
#6973=CARTESIAN_POINT ( 'NONE',  ( 50.00000000000000000, 10.00000000000000000, 0.000000000000000000 ) ) ;
#6987=SHAPE_REPRESENTATION ( 'V_bar', ( #1587 ), #1923 ) ;
#7007=DIRECTION ( 'NONE',  ( 0.000000000000000000, 1.000000000000000000, 0.000000000000000000 ) ) ;
#7043=MECHANICAL_DESIGN_GEOMETRIC_PRESENTATION_REPRESENTATION('',(#3061),#5454);
#7057=CARTESIAN_POINT ( 'NONE',  ( 60.00000000000000711, -10.00000000000000000, 60.00000000000000000 ) ) ;
#7081=COLOUR_RGB ( '', 0.66274510, 0.83137255, 0.94901961) ;
#7084=CARTESIAN_POINT ( 'NONE',  ( 0.000000000000000000, 0.000000000000000000, 0.000000000000000000 ) ) ;
#7090=VECTOR ( 'NONE', #4154, 1000.000000000000000 ) ;
#7134=VERTEX_POINT ( 'NONE', #4052 ) ;
#7144=DIRECTION ( 'NONE',  ( 1.000000000000000000, 0.000000000000000000, 0.000000000000000000 ) ) ;
#7193=CARTESIAN_POINT ( 'NONE',  ( 52.00000000000000711, -8.000000000000000000, -8.000000000000000000 ) ) ;
#7194=ADVANCED_FACE ( 'NONE', ( #5597 ), #4880, .T. ) ;
#7204=EDGE_LOOP ( 'NONE', ( #817, #421, #1162, #3806 ) ) ;
#7211=DIRECTION ( 'NONE',  ( 1.000000000000000000, -0.000000000000000000, -0.000000000000000000 ) ) ;
#7222=FACE_OUTER_BOUND ( 'NONE', #3037, .T. ) ;
#7234=EDGE_CURVE ( 'NONE', #4539, #4068, #2121, .T. ) ;
#7304=FACE_OUTER_BOUND ( 'NONE', #4690, .T. ) ;
#7324=AXIS2_PLACEMENT_3D ( 'NONE', #5309, #7829, #299 ) ;
#7339=FACE_OUTER_BOUND ( 'NONE', #4257, .T. ) ;
#7344=ADVANCED_FACE ( 'NONE', ( #5065, #1475 ), #7814, .T. ) ;
#7356=DIRECTION ( 'NONE',  ( -1.000000000000000000, 0.000000000000000000, 0.000000000000000000 ) ) ;
#7359=DIRECTION ( 'NONE',  ( -0.000000000000000000, 1.000000000000000000, -0.000000000000000000 ) ) ;
#7376=ORIENTED_EDGE ( 'NONE', *, *, #556, .F. ) ;
#7407=ADVANCED_FACE ( 'NONE', ( #4125 ), #6603, .F. ) ;
#7420=DIRECTION ( 'NONE',  ( 0.000000000000000000, 1.000000000000000000, 0.000000000000000000 ) ) ;
#7439=ORIENTED_EDGE ( 'NONE', *, *, #1750, .T. ) ;
#7447=UNCERTAINTY_MEASURE_WITH_UNIT (LENGTH_MEASURE( 1.000000000000000082E-05 ), #6567, 'distance_accuracy_value', 'NONE');
#7455=EDGE_CURVE ( 'NONE', #931, #3615, #5872, .T. ) ;
#7456=DIRECTION ( 'NONE',  ( 1.000000000000000000, 0.000000000000000000, 0.000000000000000000 ) ) ;
#7484=ORIENTED_EDGE ( 'NONE', *, *, #1983, .T. ) ;
#7521=ORIENTED_EDGE ( 'NONE', *, *, #7847, .T. ) ;
#7548=CARTESIAN_POINT ( 'NONE',  ( 60.00000000000000711, 9.332579536216795825E-15, 53.34999999999998721 ) ) ;
#7577=LINE ( 'NONE', #1843, #1709 ) ;
#7580=CARTESIAN_POINT ( 'NONE',  ( 55.00000000000000000, -8.000000000000001776, -2.849999999999991651 ) ) ;
#7595=ORIENTED_EDGE ( 'NONE', *, *, #2137, .T. ) ;
#7603=AXIS2_PLACEMENT_3D ( 'NONE', #1663, #407, #2947 ) ;
#7628=FILL_AREA_STYLE_COLOUR ( '', #2537 ) ;
#7632=LINE ( 'NONE', #4477, #5843 ) ;
#7659=ORIENTED_EDGE ( 'NONE', *, *, #3808, .F. ) ;
#7673=VECTOR ( 'NONE', #4779, 1000.000000000000000 ) ;
#7695=DIRECTION ( 'NONE',  ( 0.000000000000000000, 1.000000000000000000, 0.000000000000000000 ) ) ;
#7720=DIRECTION ( 'NONE',  ( 0.000000000000000000, 0.000000000000000000, -1.000000000000000000 ) ) ;
#7738=ORIENTED_EDGE ( 'NONE', *, *, #4117, .T. ) ;
#7751=ORIENTED_EDGE ( 'NONE', *, *, #2862, .T. ) ;
#7762=CARTESIAN_POINT ( 'NONE',  ( 58.00000000000000000, 8.000000000000000000, 0.000000000000000000 ) ) ;
#7766=SHAPE_DEFINITION_REPRESENTATION ( #4313, #6987 ) ;
#7781=CARTESIAN_POINT ( 'NONE',  ( 50.00000000000000000, -10.00000000000000000, 0.000000000000000000 ) ) ;
#7801=EDGE_CURVE ( 'NONE', #6597, #7134, #5518, .T. ) ;
#7814=PLANE ( 'NONE',  #6235 ) ;
#7824=VECTOR ( 'NONE', #8116, 1000.000000000000000 ) ;
#7829=DIRECTION ( 'NONE',  ( 1.000000000000000000, -0.000000000000000000, -0.000000000000000000 ) ) ;
#7838=EDGE_LOOP ( 'NONE', ( #4067, #981, #4542, #2995 ) ) ;
#7847=EDGE_CURVE ( 'NONE', #4432, #3047, #4632, .T. ) ;
#7857=CARTESIAN_POINT ( 'NONE',  ( 60.00000000000000711, 9.534646258076108189E-15, 56.64999999999996305 ) ) ;
#7859=EDGE_CURVE ( 'NONE', #7134, #5096, #4720, .T. ) ;
#7868=LINE ( 'NONE', #7905, #2361 ) ;
#7869=DIRECTION ( 'NONE',  ( 0.000000000000000000, 0.000000000000000000, 1.000000000000000000 ) ) ;
#7895=VECTOR ( 'NONE', #7359, 1000.000000000000000 ) ;
#7901=ORIENTED_EDGE ( 'NONE', *, *, #2520, .F. ) ;
#7905=CARTESIAN_POINT ( 'NONE',  ( 60.00000000000000711, -10.00000000000000000, 60.00000000000000000 ) ) ;
#7942=UNCERTAINTY_MEASURE_WITH_UNIT (LENGTH_MEASURE( 1.000000000000000082E-05 ), #5802, 'distance_accuracy_value', 'NONE');
#7945=VECTOR ( 'NONE', #3560, 1000.000000000000000 ) ;
#7961=DIRECTION ( 'NONE',  ( 0.000000000000000000, -0.000000000000000000, 1.000000000000000000 ) ) ;
#7999=ORIENTED_EDGE ( 'NONE', *, *, #4889, .T. ) ;
#8025=LINE ( 'NONE', #4342, #7824 ) ;
#8038=ORIENTED_EDGE ( 'NONE', *, *, #4204, .F. ) ;
#8044=DIRECTION ( 'NONE',  ( -0.000000000000000000, -0.000000000000000000, -1.000000000000000000 ) ) ;
#8061=ORIENTED_EDGE ( 'NONE', *, *, #556, .T. ) ;
#8116=DIRECTION ( 'NONE',  ( -1.000000000000000000, 0.000000000000000000, 0.000000000000000000 ) ) ;
#8148=VERTEX_POINT ( 'NONE', #5915 ) ;
ENDSEC;
END-ISO-10303-21;
